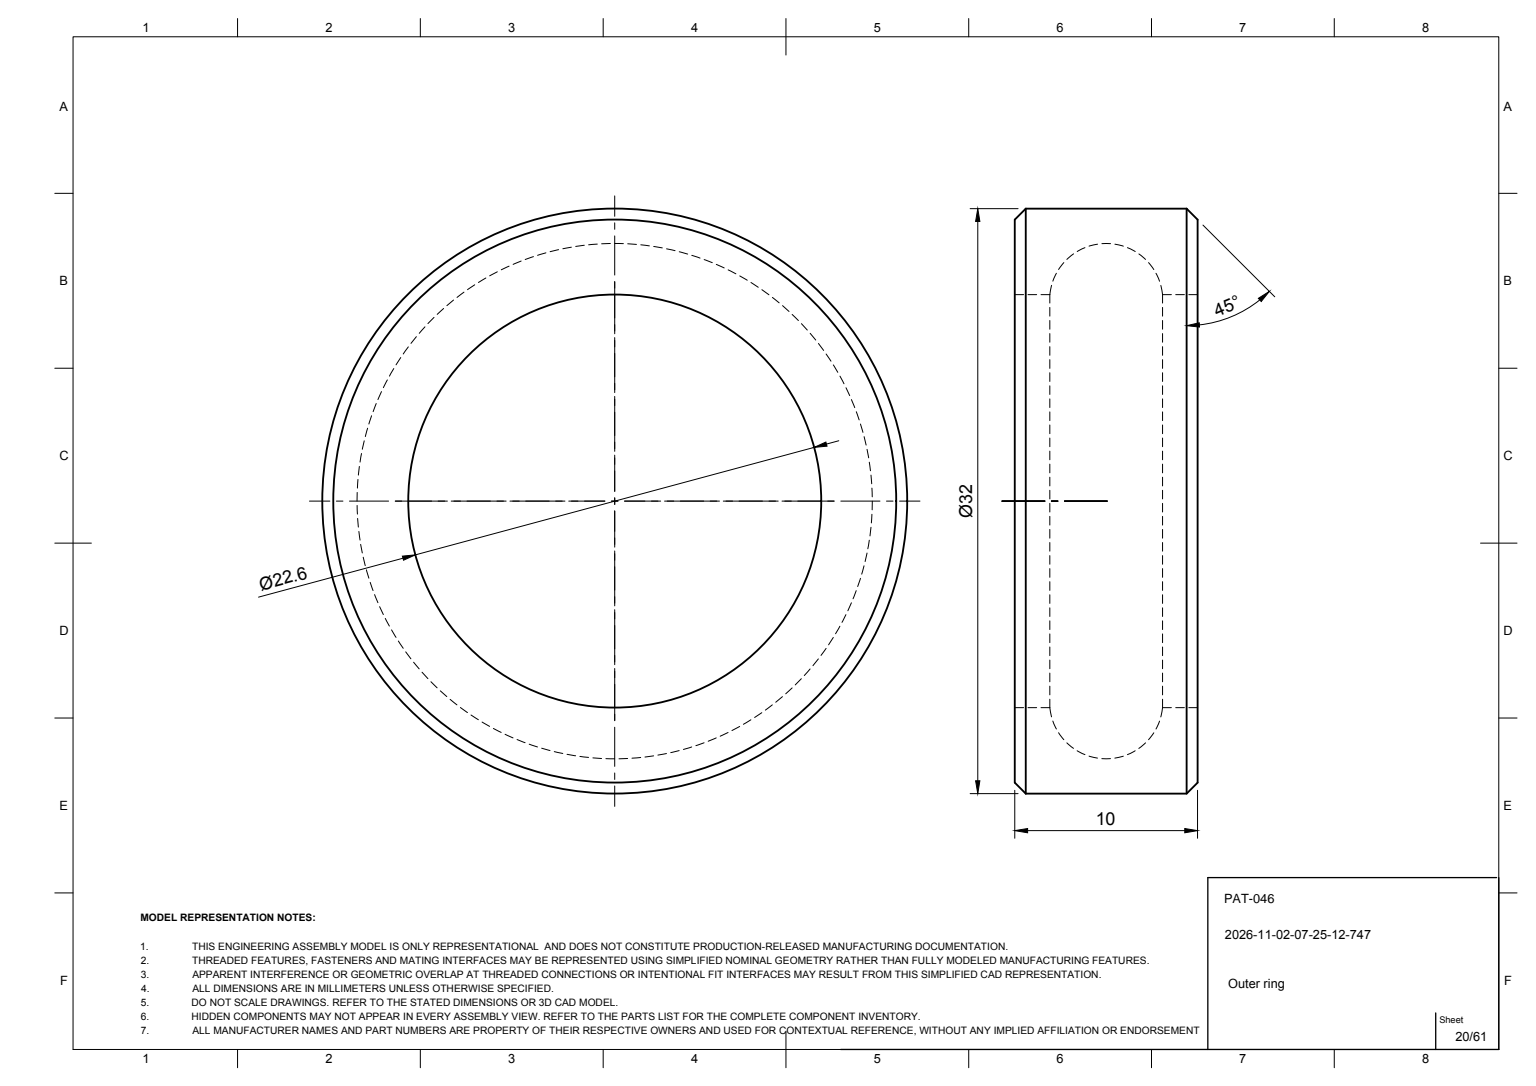
ISO-10303-21;
HEADER;
/* Generated by software containing ST-Developer
 * from STEP Tools, Inc. (www.steptools.com) 
 */

FILE_DESCRIPTION(
/* description */ ('Gear mesh backlash fixture'),
/* implementation_level */ '2;1');

FILE_NAME(
/* name */ 'Outer ring.step',
/* time_stamp */ '2026-10-28T03:26:00-07:00',
/* author */ (''),
/* organization */ (''),
/* preprocessor_version */ 'ST-DEVELOPER v20.2',
/* originating_system */ 'Autodesk Translation Framework v15.17.0.0',
/* authorisation */ '');

FILE_SCHEMA (('AUTOMOTIVE_DESIGN { 1 0 10303 214 3 1 1 }'));
ENDSEC;

DATA;
#10=MECHANICAL_DESIGN_GEOMETRIC_PRESENTATION_REPRESENTATION('',(#1029),#57900);
#761=CONICAL_SURFACE('',#14529,1.57,0.785398163397449);
#762=CONICAL_SURFACE('',#14533,1.57,0.785398163397449);
#781=TOROIDAL_SURFACE('',#14518,1.1,0.309556);
#929=SHAPE_REPRESENTATION_RELATIONSHIP('SRR','None',#58125,#979);
#979=ADVANCED_BREP_SHAPE_REPRESENTATION('',(#1094),#57858);
#1029=STYLED_ITEM('',(#58465),#1094);
#1094=MANIFOLD_SOLID_BREP('Body1',#13589);
#1219=FACE_BOUND('',#2692,.T.);
#1220=FACE_BOUND('',#2697,.T.);
#1415=PLANE('',#14526);
#1416=PLANE('',#14535);
#1848=FACE_OUTER_BOUND('',#2689,.T.);
#1849=FACE_OUTER_BOUND('',#2690,.T.);
#1850=FACE_OUTER_BOUND('',#2691,.T.);
#1851=FACE_OUTER_BOUND('',#2693,.T.);
#1852=FACE_OUTER_BOUND('',#2694,.T.);
#1853=FACE_OUTER_BOUND('',#2695,.T.);
#1854=FACE_OUTER_BOUND('',#2696,.T.);
#1855=FACE_OUTER_BOUND('',#2698,.T.);
#2689=EDGE_LOOP('',(#9579,#9580,#9581,#9582,#9583,#9584));
#2690=EDGE_LOOP('',(#9585,#9586,#9587,#9588,#9589));
#2691=EDGE_LOOP('',(#9590));
#2692=EDGE_LOOP('',(#9591));
#2693=EDGE_LOOP('',(#9592,#9593,#9594,#9595));
#2694=EDGE_LOOP('',(#9596,#9597,#9598,#9599));
#2695=EDGE_LOOP('',(#9600,#9601,#9602,#9603));
#2696=EDGE_LOOP('',(#9604));
#2697=EDGE_LOOP('',(#9605));
#2698=EDGE_LOOP('',(#9606,#9607,#9608,#9609,#9610));
#3602=LINE('',#20090,#4491);
#3603=LINE('',#20099,#4492);
#3604=LINE('',#20103,#4493);
#3605=LINE('',#20107,#4494);
#3606=LINE('',#20110,#4495);
#4491=VECTOR('',#16431,1.129765);
#4492=VECTOR('',#16442,1.57);
#4493=VECTOR('',#16447,1.6);
#4494=VECTOR('',#16452,1.57);
#4495=VECTOR('',#16457,1.129765);
#5341=CIRCLE('',#14519,1.129765);
#5342=CIRCLE('',#14520,1.129765);
#5343=CIRCLE('',#14521,0.309556);
#5344=CIRCLE('',#14522,1.129765);
#5345=CIRCLE('',#14523,1.129765);
#5346=CIRCLE('',#14525,1.129765);
#5347=CIRCLE('',#14527,1.54);
#5348=CIRCLE('',#14528,1.129765);
#5349=CIRCLE('',#14530,1.6);
#5350=CIRCLE('',#14532,1.6);
#5351=CIRCLE('',#14534,1.54);
#6009=VERTEX_POINT('',#20078);
#6010=VERTEX_POINT('',#20079);
#6011=VERTEX_POINT('',#20082);
#6012=VERTEX_POINT('',#20084);
#6013=VERTEX_POINT('',#20088);
#6014=VERTEX_POINT('',#20092);
#6015=VERTEX_POINT('',#20094);
#6016=VERTEX_POINT('',#20097);
#6017=VERTEX_POINT('',#20101);
#6018=VERTEX_POINT('',#20105);
#7376=EDGE_CURVE('',#6009,#6010,#5341,.T.);
#7377=EDGE_CURVE('',#6010,#6009,#5342,.T.);
#7378=EDGE_CURVE('',#6010,#6011,#5343,.T.);
#7379=EDGE_CURVE('',#6012,#6011,#5344,.T.);
#7380=EDGE_CURVE('',#6011,#6012,#5345,.T.);
#7381=EDGE_CURVE('',#6013,#6013,#5346,.T.);
#7382=EDGE_CURVE('',#6013,#6012,#3602,.T.);
#7383=EDGE_CURVE('',#6014,#6014,#5347,.T.);
#7384=EDGE_CURVE('',#6015,#6015,#5348,.T.);
#7385=EDGE_CURVE('',#6016,#6016,#5349,.T.);
#7386=EDGE_CURVE('',#6016,#6014,#3603,.T.);
#7387=EDGE_CURVE('',#6017,#6017,#5350,.T.);
#7388=EDGE_CURVE('',#6017,#6016,#3604,.T.);
#7389=EDGE_CURVE('',#6018,#6018,#5351,.T.);
#7390=EDGE_CURVE('',#6018,#6017,#3605,.T.);
#7391=EDGE_CURVE('',#6009,#6015,#3606,.T.);
#9579=ORIENTED_EDGE('',*,*,#7376,.F.);
#9580=ORIENTED_EDGE('',*,*,#7377,.F.);
#9581=ORIENTED_EDGE('',*,*,#7378,.T.);
#9582=ORIENTED_EDGE('',*,*,#7379,.F.);
#9583=ORIENTED_EDGE('',*,*,#7380,.F.);
#9584=ORIENTED_EDGE('',*,*,#7378,.F.);
#9585=ORIENTED_EDGE('',*,*,#7381,.T.);
#9586=ORIENTED_EDGE('',*,*,#7382,.T.);
#9587=ORIENTED_EDGE('',*,*,#7379,.T.);
#9588=ORIENTED_EDGE('',*,*,#7380,.T.);
#9589=ORIENTED_EDGE('',*,*,#7382,.F.);
#9590=ORIENTED_EDGE('',*,*,#7383,.F.);
#9591=ORIENTED_EDGE('',*,*,#7384,.T.);
#9592=ORIENTED_EDGE('',*,*,#7385,.F.);
#9593=ORIENTED_EDGE('',*,*,#7386,.T.);
#9594=ORIENTED_EDGE('',*,*,#7383,.T.);
#9595=ORIENTED_EDGE('',*,*,#7386,.F.);
#9596=ORIENTED_EDGE('',*,*,#7387,.F.);
#9597=ORIENTED_EDGE('',*,*,#7388,.T.);
#9598=ORIENTED_EDGE('',*,*,#7385,.T.);
#9599=ORIENTED_EDGE('',*,*,#7388,.F.);
#9600=ORIENTED_EDGE('',*,*,#7389,.F.);
#9601=ORIENTED_EDGE('',*,*,#7390,.T.);
#9602=ORIENTED_EDGE('',*,*,#7387,.T.);
#9603=ORIENTED_EDGE('',*,*,#7390,.F.);
#9604=ORIENTED_EDGE('',*,*,#7389,.T.);
#9605=ORIENTED_EDGE('',*,*,#7381,.F.);
#9606=ORIENTED_EDGE('',*,*,#7376,.T.);
#9607=ORIENTED_EDGE('',*,*,#7377,.T.);
#9608=ORIENTED_EDGE('',*,*,#7391,.T.);
#9609=ORIENTED_EDGE('',*,*,#7384,.F.);
#9610=ORIENTED_EDGE('',*,*,#7391,.F.);
#12651=CYLINDRICAL_SURFACE('',#14524,1.129765);
#12652=CYLINDRICAL_SURFACE('',#14531,1.6);
#12653=CYLINDRICAL_SURFACE('',#14536,1.129765);
#12965=ADVANCED_FACE('',(#1848),#781,.F.);
#12966=ADVANCED_FACE('',(#1849),#12651,.F.);
#12967=ADVANCED_FACE('',(#1850,#1219),#1415,.T.);
#12968=ADVANCED_FACE('',(#1851),#761,.T.);
#12969=ADVANCED_FACE('',(#1852),#12652,.T.);
#12970=ADVANCED_FACE('',(#1853),#762,.T.);
#12971=ADVANCED_FACE('',(#1854,#1220),#1416,.T.);
#12972=ADVANCED_FACE('',(#1855),#12653,.F.);
#13589=CLOSED_SHELL('',(#12965,#12966,#12967,#12968,#12969,#12970,#12971,
#12972));
#14517=AXIS2_PLACEMENT_3D('',#20076,#16413,#16414);
#14518=AXIS2_PLACEMENT_3D('',#20077,#16415,#16416);
#14519=AXIS2_PLACEMENT_3D('',#20080,#16417,#16418);
#14520=AXIS2_PLACEMENT_3D('',#20081,#16419,#16420);
#14521=AXIS2_PLACEMENT_3D('',#20083,#16421,#16422);
#14522=AXIS2_PLACEMENT_3D('',#20085,#16423,#16424);
#14523=AXIS2_PLACEMENT_3D('',#20086,#16425,#16426);
#14524=AXIS2_PLACEMENT_3D('',#20087,#16427,#16428);
#14525=AXIS2_PLACEMENT_3D('',#20089,#16429,#16430);
#14526=AXIS2_PLACEMENT_3D('',#20091,#16432,#16433);
#14527=AXIS2_PLACEMENT_3D('',#20093,#16434,#16435);
#14528=AXIS2_PLACEMENT_3D('',#20095,#16436,#16437);
#14529=AXIS2_PLACEMENT_3D('',#20096,#16438,#16439);
#14530=AXIS2_PLACEMENT_3D('',#20098,#16440,#16441);
#14531=AXIS2_PLACEMENT_3D('',#20100,#16443,#16444);
#14532=AXIS2_PLACEMENT_3D('',#20102,#16445,#16446);
#14533=AXIS2_PLACEMENT_3D('',#20104,#16448,#16449);
#14534=AXIS2_PLACEMENT_3D('',#20106,#16450,#16451);
#14535=AXIS2_PLACEMENT_3D('',#20108,#16453,#16454);
#14536=AXIS2_PLACEMENT_3D('',#20109,#16455,#16456);
#16413=DIRECTION('axis',(0.,0.,1.));
#16414=DIRECTION('refdir',(1.,0.,0.));
#16415=DIRECTION('center_axis',(0.,-1.,0.));
#16416=DIRECTION('ref_axis',(0.,0.,-1.));
#16417=DIRECTION('center_axis',(0.,-1.,0.));
#16418=DIRECTION('ref_axis',(1.,0.,0.));
#16419=DIRECTION('center_axis',(0.,-1.,0.));
#16420=DIRECTION('ref_axis',(1.,0.,0.));
#16421=DIRECTION('center_axis',(1.,0.,1.22464679914735E-16));
#16422=DIRECTION('ref_axis',(-1.22464679914735E-16,0.,1.));
#16423=DIRECTION('center_axis',(0.,1.,0.));
#16424=DIRECTION('ref_axis',(1.,0.,0.));
#16425=DIRECTION('center_axis',(0.,1.,0.));
#16426=DIRECTION('ref_axis',(1.,0.,0.));
#16427=DIRECTION('center_axis',(0.,-1.,0.));
#16428=DIRECTION('ref_axis',(1.,0.,0.));
#16429=DIRECTION('center_axis',(0.,-1.,0.));
#16430=DIRECTION('ref_axis',(1.,0.,0.));
#16431=DIRECTION('',(0.,1.,0.));
#16432=DIRECTION('center_axis',(0.,1.,0.));
#16433=DIRECTION('ref_axis',(0.,0.,1.));
#16434=DIRECTION('center_axis',(0.,-1.,0.));
#16435=DIRECTION('ref_axis',(1.,0.,0.));
#16436=DIRECTION('center_axis',(0.,-1.,0.));
#16437=DIRECTION('ref_axis',(1.,0.,0.));
#16438=DIRECTION('center_axis',(0.,-1.,0.));
#16439=DIRECTION('ref_axis',(1.,0.,0.));
#16440=DIRECTION('center_axis',(0.,-1.,0.));
#16441=DIRECTION('ref_axis',(1.,0.,0.));
#16442=DIRECTION('',(0.707106781186548,0.707106781186547,8.65956056235494E-17));
#16443=DIRECTION('center_axis',(0.,-1.,0.));
#16444=DIRECTION('ref_axis',(1.,0.,0.));
#16445=DIRECTION('center_axis',(0.,-1.,0.));
#16446=DIRECTION('ref_axis',(1.,0.,0.));
#16447=DIRECTION('',(0.,1.,0.));
#16448=DIRECTION('center_axis',(0.,1.,0.));
#16449=DIRECTION('ref_axis',(1.,0.,0.));
#16450=DIRECTION('center_axis',(0.,-1.,0.));
#16451=DIRECTION('ref_axis',(1.,0.,0.));
#16452=DIRECTION('',(-0.707106781186548,0.707106781186547,-8.65956056235494E-17));
#16453=DIRECTION('center_axis',(0.,-1.,0.));
#16454=DIRECTION('ref_axis',(0.,0.,-1.));
#16455=DIRECTION('center_axis',(0.,-1.,0.));
#16456=DIRECTION('ref_axis',(1.,0.,0.));
#16457=DIRECTION('',(0.,1.,0.));
#20076=CARTESIAN_POINT('',(0.,0.,0.));
#20077=CARTESIAN_POINT('Origin',(0.,0.,0.));
#20078=CARTESIAN_POINT('',(-1.129765,0.308121667383195,-1.38356309103871E-16));
#20079=CARTESIAN_POINT('',(-1.38356309103871E-16,0.308121667383195,1.129765));
#20080=CARTESIAN_POINT('Origin',(0.,0.308121667383195,0.));
#20081=CARTESIAN_POINT('Origin',(0.,0.308121667383195,0.));
#20082=CARTESIAN_POINT('',(-1.38356309103871E-16,-0.308121667383195,1.129765));
#20083=CARTESIAN_POINT('Origin',(-1.34711147906209E-16,0.,1.1));
#20084=CARTESIAN_POINT('',(-1.129765,-0.308121667383195,1.38356309103871E-16));
#20085=CARTESIAN_POINT('Origin',(0.,-0.308121667383195,0.));
#20086=CARTESIAN_POINT('Origin',(0.,-0.308121667383195,0.));
#20087=CARTESIAN_POINT('Origin',(0.,0.,0.));
#20088=CARTESIAN_POINT('',(-1.129765,-0.5,-1.38356309103871E-16));
#20089=CARTESIAN_POINT('Origin',(0.,-0.5,0.));
#20090=CARTESIAN_POINT('',(-1.129765,0.,-1.38356309103871E-16));
#20091=CARTESIAN_POINT('Origin',(1.54,0.5,0.));
#20092=CARTESIAN_POINT('',(-1.54,0.5,-1.88595607068692E-16));
#20093=CARTESIAN_POINT('Origin',(0.,0.5,0.));
#20094=CARTESIAN_POINT('',(-1.129765,0.5,-1.38356309103871E-16));
#20095=CARTESIAN_POINT('Origin',(0.,0.5,0.));
#20096=CARTESIAN_POINT('Origin',(0.,0.47,0.));
#20097=CARTESIAN_POINT('',(-1.6,0.44,-1.95943487863577E-16));
#20098=CARTESIAN_POINT('Origin',(0.,0.44,0.));
#20099=CARTESIAN_POINT('',(-1.57,0.47,-1.92269547466134E-16));
#20100=CARTESIAN_POINT('Origin',(0.,0.,0.));
#20101=CARTESIAN_POINT('',(-1.6,-0.44,-1.95943487863577E-16));
#20102=CARTESIAN_POINT('Origin',(0.,-0.44,0.));
#20103=CARTESIAN_POINT('',(-1.6,0.,-1.95943487863577E-16));
#20104=CARTESIAN_POINT('Origin',(0.,-0.47,0.));
#20105=CARTESIAN_POINT('',(-1.54,-0.5,-1.88595607068692E-16));
#20106=CARTESIAN_POINT('Origin',(0.,-0.5,0.));
#20107=CARTESIAN_POINT('',(-1.57,-0.47,-1.92269547466134E-16));
#20108=CARTESIAN_POINT('Origin',(1.129765,-0.5,0.));
#20109=CARTESIAN_POINT('Origin',(0.,0.,0.));
#20110=CARTESIAN_POINT('',(-1.129765,0.,-1.38356309103871E-16));
#57799=UNCERTAINTY_MEASURE_WITH_UNIT(LENGTH_MEASURE(0.001),#57901,
'DISTANCE_ACCURACY_VALUE',
'Maximum model space distance between geometric entities at asserted c
onnectivities');
#57841=UNCERTAINTY_MEASURE_WITH_UNIT(LENGTH_MEASURE(0.001),#57901,
'DISTANCE_ACCURACY_VALUE',
'Maximum model space distance between geometric entities at asserted c
onnectivities');
#57858=(
GEOMETRIC_REPRESENTATION_CONTEXT(3)
GLOBAL_UNCERTAINTY_ASSIGNED_CONTEXT((#57799))
GLOBAL_UNIT_ASSIGNED_CONTEXT((#57901,#57903,#57904))
REPRESENTATION_CONTEXT('','3D')
);
#57900=(
GEOMETRIC_REPRESENTATION_CONTEXT(3)
GLOBAL_UNCERTAINTY_ASSIGNED_CONTEXT((#57841))
GLOBAL_UNIT_ASSIGNED_CONTEXT((#57901,#57903,#57904))
REPRESENTATION_CONTEXT('','3D')
);
#57901=(
LENGTH_UNIT()
NAMED_UNIT(*)
SI_UNIT(.CENTI.,.METRE.)
);
#57903=(
NAMED_UNIT(*)
PLANE_ANGLE_UNIT()
SI_UNIT($,.RADIAN.)
);
#57904=(
NAMED_UNIT(*)
SI_UNIT($,.STERADIAN.)
SOLID_ANGLE_UNIT()
);
#57921=SHAPE_DEFINITION_REPRESENTATION(#57979,#58125);
#57979=PRODUCT_DEFINITION_SHAPE('',$,#58184);
#58125=SHAPE_REPRESENTATION('',(#14517),#57858);
#58167=PRODUCT_DEFINITION_CONTEXT('part definition',#58343,'design');
#58184=PRODUCT_DEFINITION('Outer ring','Outer ring',#58242,#58167);
#58242=PRODUCT_DEFINITION_FORMATION('',$,#58361);
#58343=APPLICATION_CONTEXT(
'Core Data for Automotive Mechanical Design Process');
#58344=PRODUCT_CONTEXT('part definition',#58343,'mechanical');
#58361=PRODUCT('Outer ring','Outer ring','Outer ring',(#58344));
#58459=COLOUR_RGB('Grey',0.48,0.52,0.57);
#58460=FILL_AREA_STYLE_COLOUR('',#58459);
#58461=FILL_AREA_STYLE('',(#58460));
#58462=SURFACE_STYLE_FILL_AREA(#58461);
#58463=SURFACE_SIDE_STYLE('',(#58462));
#58464=SURFACE_STYLE_USAGE(.BOTH.,#58463);
#58465=PRESENTATION_STYLE_ASSIGNMENT((#58464));
ENDSEC;
END-ISO-10303-21;
